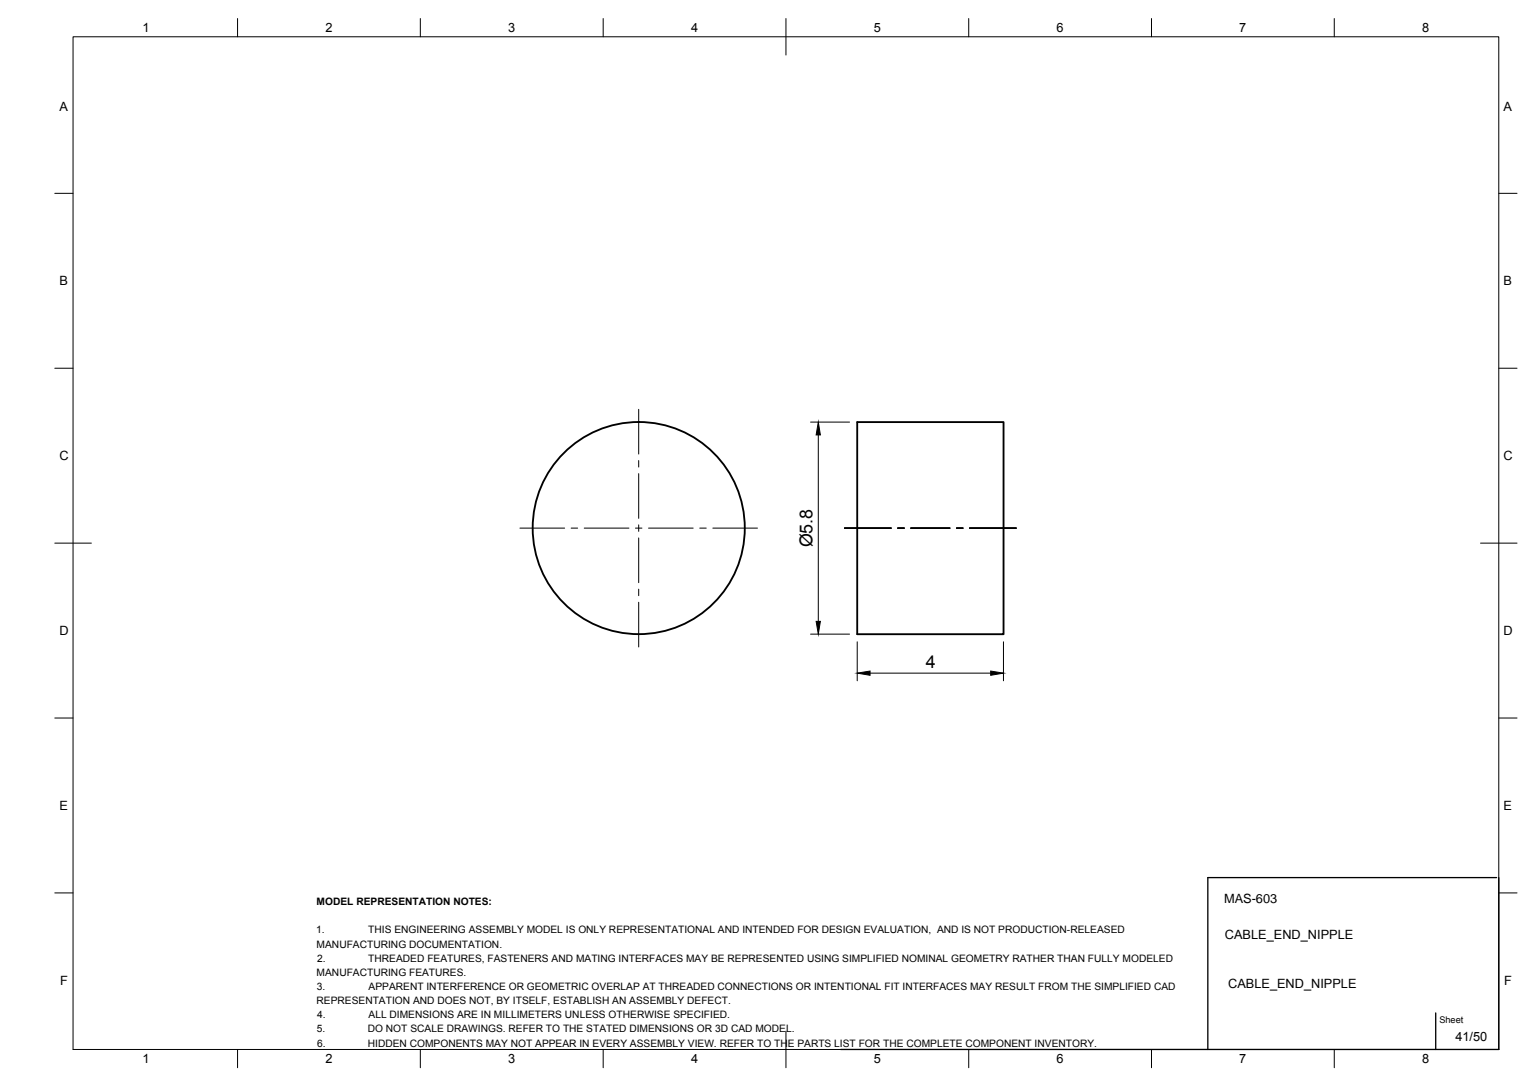
ISO-10303-21;
HEADER;
FILE_DESCRIPTION((''),'2;1');
FILE_NAME('CABLE_END_NIPPLE.step','2026-10-01T22:06:14-07:00',(''),(''),'','','');
FILE_SCHEMA (('AUTOMOTIVE_DESIGN { 1 0 10303 214 3 1 1 }'));
ENDSEC;
DATA;
#10=MECHANICAL_DESIGN_GEOMETRIC_PRESENTATION_REPRESENTATION('',(#1015),#50440);
#921=SHAPE_REPRESENTATION_RELATIONSHIP('SRR','None',#50654,#966) ;
#966=ADVANCED_BREP_SHAPE_REPRESENTATION('',(#1069),#50423) ;
#1015=STYLED_ITEM('',(#50887),#1069) ;
#1069=MANIFOLD_SOLID_BREP('CABLE_END_NIPPLE',#28691) ;
#2240=PLANE('',#31061) ;
#2241=PLANE('',#31062) ;
#3469=FACE_OUTER_BOUND('',#5290,.T.) ;
#3470=FACE_OUTER_BOUND('',#5291,.T.) ;
#3471=FACE_OUTER_BOUND('',#5292,.T.) ;
#5290=EDGE_LOOP('',(#24283,#24284,#24285,#24286)) ;
#5291=EDGE_LOOP('',(#24287)) ;
#5292=EDGE_LOOP('',(#24288)) ;
#7899=LINE('',#47507,#10371) ;
#10371=VECTOR('',#38244,0.29) ;
#11291=CIRCLE('',#31059,0.29) ;
#11292=CIRCLE('',#31060,0.29) ;
#13749=VERTEX_POINT('',#47504) ;
#13750=VERTEX_POINT('',#47506) ;
#17407=EDGE_CURVE('',#13749,#13749,#11291,.T.) ;
#17408=EDGE_CURVE('',#13749,#13750,#7899,.T.) ;
#17409=EDGE_CURVE('',#13750,#13750,#11292,.T.) ;
#24283=ORIENTED_EDGE('',*,*,#17407,.F.) ;
#24284=ORIENTED_EDGE('',*,*,#17408,.T.) ;
#24285=ORIENTED_EDGE('',*,*,#17409,.F.) ;
#24286=ORIENTED_EDGE('',*,*,#17408,.F.) ;
#24287=ORIENTED_EDGE('',*,*,#17409,.T.) ;
#24288=ORIENTED_EDGE('',*,*,#17407,.T.) ;
#26893=CYLINDRICAL_SURFACE('',#31058,0.29) ;
#28204=ADVANCED_FACE('',(#3469),#26893,.T.) ;
#28205=ADVANCED_FACE('',(#3470),#2240,.T.) ;
#28206=ADVANCED_FACE('',(#3471),#2241,.T.) ;
#28691=CLOSED_SHELL('',(#28204,#28205,#28206)) ;
#31057=AXIS2_PLACEMENT_3D('',#47502,#38238,#38239) ;
#31058=AXIS2_PLACEMENT_3D('',#47503,#38240,#38241) ;
#31059=AXIS2_PLACEMENT_3D('',#47505,#38242,#38243) ;
#31060=AXIS2_PLACEMENT_3D('',#47508,#38245,#38246) ;
#31061=AXIS2_PLACEMENT_3D('',#47509,#38247,#38248) ;
#31062=AXIS2_PLACEMENT_3D('',#47510,#38249,#38250) ;
#38238=DIRECTION('axis',(0.,0.,1.)) ;
#38239=DIRECTION('refdir',(1.,0.,0.)) ;
#38240=DIRECTION('center_axis',(0.,0.,1.)) ;
#38241=DIRECTION('ref_axis',(1.,0.,0.)) ;
#38242=DIRECTION('center_axis',(0.,0.,1.)) ;
#38243=DIRECTION('ref_axis',(1.,0.,0.)) ;
#38244=DIRECTION('',(0.,0.,-1.)) ;
#38245=DIRECTION('center_axis',(0.,0.,-1.)) ;
#38246=DIRECTION('ref_axis',(1.,0.,0.)) ;
#38247=DIRECTION('center_axis',(0.,0.,-1.)) ;
#38248=DIRECTION('ref_axis',(-1.,0.,0.)) ;
#38249=DIRECTION('center_axis',(0.,0.,1.)) ;
#38250=DIRECTION('ref_axis',(1.,0.,0.)) ;
#47502=CARTESIAN_POINT('',(0.,0.,0.)) ;
#47503=CARTESIAN_POINT('Origin',(-13.,0.,42.6)) ;
#47504=CARTESIAN_POINT('',(-13.29,-3.55147571752732E-17,42.8)) ;
#47505=CARTESIAN_POINT('Origin',(-13.,0.,42.8)) ;
#47506=CARTESIAN_POINT('',(-13.29,-3.55147571752732E-17,42.4)) ;
#47507=CARTESIAN_POINT('',(-13.29,-3.55147571752732E-17,42.6)) ;
#47508=CARTESIAN_POINT('Origin',(-13.,0.,42.4)) ;
#47509=CARTESIAN_POINT('Origin',(-13.,0.,42.4)) ;
#47510=CARTESIAN_POINT('Origin',(-13.,0.,42.8)) ;
#50370=UNCERTAINTY_MEASURE_WITH_UNIT(LENGTH_MEASURE(0.001),#50441,
'DISTANCE_ACCURACY_VALUE',
'Maximum model space distance between geometric entities at asserted c
onnectivities') ;
#50387=UNCERTAINTY_MEASURE_WITH_UNIT(LENGTH_MEASURE(0.001),#50441,
'DISTANCE_ACCURACY_VALUE',
'Maximum model space distance between geometric entities at asserted c
onnectivities') ;
#50423=(
GEOMETRIC_REPRESENTATION_CONTEXT(3)
GLOBAL_UNCERTAINTY_ASSIGNED_CONTEXT((#50370))
GLOBAL_UNIT_ASSIGNED_CONTEXT((#50441,#50443,#50444))
REPRESENTATION_CONTEXT('','3D')
) ;
#50440=(
GEOMETRIC_REPRESENTATION_CONTEXT(3)
GLOBAL_UNCERTAINTY_ASSIGNED_CONTEXT((#50387))
GLOBAL_UNIT_ASSIGNED_CONTEXT((#50441,#50443,#50444))
REPRESENTATION_CONTEXT('','3D')
) ;
#50441=(
LENGTH_UNIT()
NAMED_UNIT(*)
SI_UNIT(.CENTI.,.METRE.)
) ;
#50443=(
NAMED_UNIT(*)
PLANE_ANGLE_UNIT()
SI_UNIT($,.RADIAN.)
) ;
#50444=(
NAMED_UNIT(*)
SI_UNIT($,.STERADIAN.)
SOLID_ANGLE_UNIT()
) ;
#50480=SHAPE_DEFINITION_REPRESENTATION(#50556,#50654) ;
#50556=PRODUCT_DEFINITION_SHAPE('',$,#50707) ;
#50654=SHAPE_REPRESENTATION('',(#31057),#50423) ;
#50671=PRODUCT_DEFINITION_CONTEXT('part definition',#50829,'design') ;
#50707=PRODUCT_DEFINITION('CABLE_END_NIPPLE','CABLE_END_NIPPLE',
#50759,#50671) ;
#50759=PRODUCT_DEFINITION_FORMATION('',$,#50866) ;
#50829=APPLICATION_CONTEXT(
'Core Data for Automotive Mechanical Design Process') ;
#50830=PRODUCT_CONTEXT('part definition',#50829,'mechanical') ;
#50866=PRODUCT('CABLE_END_NIPPLE','CABLE_END_NIPPLE',$,(#50830)) ;
#50887=PRESENTATION_STYLE_ASSIGNMENT((#50894)) ;
#50894=SURFACE_STYLE_USAGE(.BOTH.,#50901) ;
#50901=SURFACE_SIDE_STYLE('',(#50908)) ;
#50908=SURFACE_STYLE_FILL_AREA(#50915) ;
#50915=FILL_AREA_STYLE('Brass - Polished',(#50922)) ;
#50922=FILL_AREA_STYLE_COLOUR('Brass - Polished',#50929) ;
#50929=COLOUR_RGB('Brass - Polished', 0.66274510, 0.83137255, 0.94901961) ;
ENDSEC;
END-ISO-10303-21;
